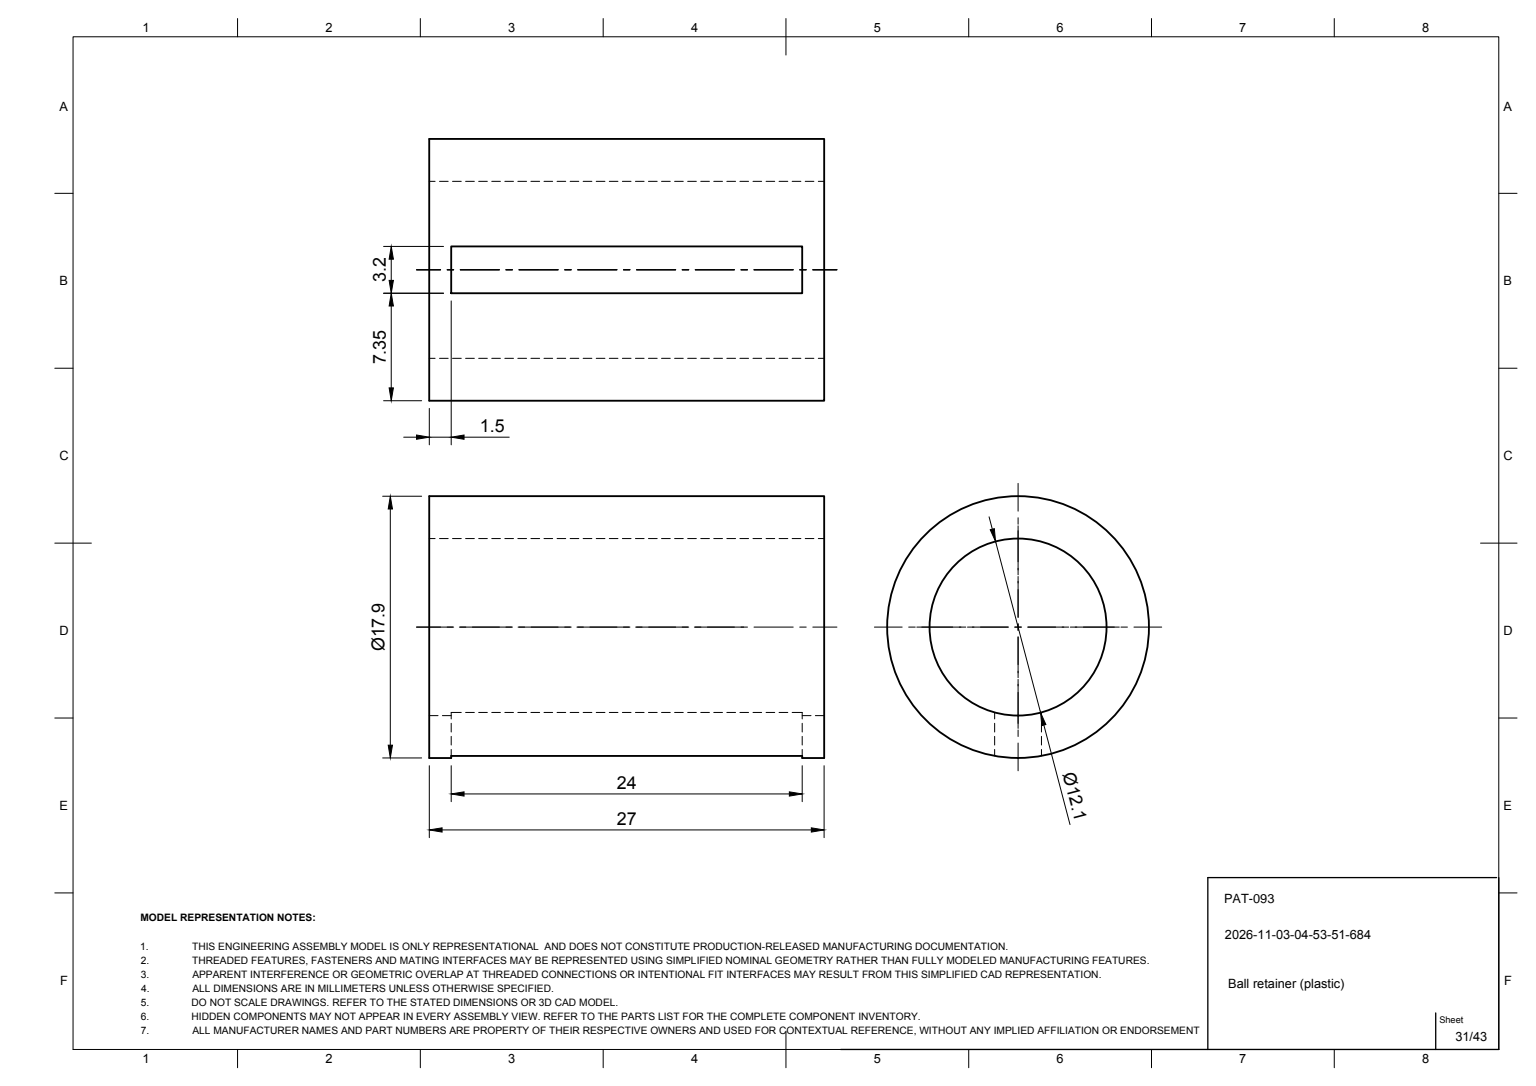
ISO-10303-21;
HEADER;
/* Generated by software containing ST-Developer
 * from STEP Tools, Inc. (www.steptools.com) 
 */

FILE_DESCRIPTION(
/* description */ ('Self-centering screw clamp'),
/* implementation_level */ '2;1');

FILE_NAME(
/* name */ 'Ball retainer (plastic).step',
/* time_stamp */ '2026-10-28T03:25:31-07:00',
/* author */ (''),
/* organization */ (''),
/* preprocessor_version */ 'ST-DEVELOPER v20.2',
/* originating_system */ 'Autodesk Translation Framework v15.17.0.0',
/* authorisation */ '');

FILE_SCHEMA (('AUTOMOTIVE_DESIGN { 1 0 10303 214 3 1 1 }'));
ENDSEC;

DATA;
#10=MECHANICAL_DESIGN_GEOMETRIC_PRESENTATION_REPRESENTATION('',(#661),#16799);
#572=SHAPE_REPRESENTATION_RELATIONSHIP('SRR','None',#17049,#613);
#613=ADVANCED_BREP_SHAPE_REPRESENTATION('',(#709),#16787);
#661=STYLED_ITEM('',(#17319),#709);
#709=MANIFOLD_SOLID_BREP('Body1',#9112);
#988=FACE_BOUND('',#2456,.T.);
#989=FACE_BOUND('',#2458,.T.);
#990=FACE_BOUND('',#2460,.T.);
#991=FACE_BOUND('',#2462,.T.);
#1211=PLANE('',#10462);
#1212=PLANE('',#10465);
#1213=PLANE('',#10466);
#1214=PLANE('',#10469);
#1215=PLANE('',#10470);
#1216=PLANE('',#10475);
#1677=FACE_OUTER_BOUND('',#2451,.T.);
#1678=FACE_OUTER_BOUND('',#2452,.T.);
#1679=FACE_OUTER_BOUND('',#2453,.T.);
#1680=FACE_OUTER_BOUND('',#2454,.T.);
#1681=FACE_OUTER_BOUND('',#2455,.T.);
#1682=FACE_OUTER_BOUND('',#2457,.T.);
#1683=FACE_OUTER_BOUND('',#2459,.T.);
#1684=FACE_OUTER_BOUND('',#2461,.T.);
#2451=EDGE_LOOP('',(#7971,#7972,#7973,#7974));
#2452=EDGE_LOOP('',(#7975,#7976,#7977,#7978));
#2453=EDGE_LOOP('',(#7979,#7980,#7981,#7982));
#2454=EDGE_LOOP('',(#7983,#7984,#7985,#7986));
#2455=EDGE_LOOP('',(#7987));
#2456=EDGE_LOOP('',(#7988));
#2457=EDGE_LOOP('',(#7989,#7990,#7991,#7992));
#2458=EDGE_LOOP('',(#7993,#7994,#7995,#7996));
#2459=EDGE_LOOP('',(#7997));
#2460=EDGE_LOOP('',(#7998));
#2461=EDGE_LOOP('',(#7999,#8000,#8001,#8002));
#2462=EDGE_LOOP('',(#8003,#8004,#8005,#8006));
#3042=LINE('',#16052,#3615);
#3043=LINE('',#16055,#3616);
#3044=LINE('',#16058,#3617);
#3045=LINE('',#16060,#3618);
#3046=LINE('',#16061,#3619);
#3047=LINE('',#16067,#3620);
#3048=LINE('',#16069,#3621);
#3049=LINE('',#16070,#3622);
#3050=LINE('',#16079,#3623);
#3051=LINE('',#16084,#3624);
#3615=VECTOR('',#12991,1.);
#3616=VECTOR('',#12994,1.);
#3617=VECTOR('',#12997,1.);
#3618=VECTOR('',#12998,1.);
#3619=VECTOR('',#12999,1.);
#3620=VECTOR('',#13006,1.);
#3621=VECTOR('',#13009,1.);
#3622=VECTOR('',#13010,1.);
#3623=VECTOR('',#13021,0.895);
#3624=VECTOR('',#13028,0.605);
#4162=CIRCLE('',#10463,0.895);
#4163=CIRCLE('',#10464,0.605);
#4164=CIRCLE('',#10467,0.895);
#4165=CIRCLE('',#10468,0.605);
#4166=CIRCLE('',#10471,0.895);
#4167=CIRCLE('',#10472,0.605);
#4168=CIRCLE('',#10474,0.895);
#4169=CIRCLE('',#10476,0.605);
#4851=VERTEX_POINT('',#16048);
#4852=VERTEX_POINT('',#16049);
#4853=VERTEX_POINT('',#16051);
#4854=VERTEX_POINT('',#16053);
#4855=VERTEX_POINT('',#16057);
#4856=VERTEX_POINT('',#16059);
#4857=VERTEX_POINT('',#16063);
#4858=VERTEX_POINT('',#16065);
#4859=VERTEX_POINT('',#16072);
#4860=VERTEX_POINT('',#16074);
#4861=VERTEX_POINT('',#16077);
#4862=VERTEX_POINT('',#16081);
#5910=EDGE_CURVE('',#4851,#4852,#4162,.T.);
#5911=EDGE_CURVE('',#4853,#4851,#3042,.T.);
#5912=EDGE_CURVE('',#4854,#4853,#4163,.T.);
#5913=EDGE_CURVE('',#4852,#4854,#3043,.T.);
#5914=EDGE_CURVE('',#4852,#4855,#3044,.T.);
#5915=EDGE_CURVE('',#4856,#4854,#3045,.T.);
#5916=EDGE_CURVE('',#4856,#4855,#3046,.T.);
#5917=EDGE_CURVE('',#4855,#4857,#4164,.T.);
#5918=EDGE_CURVE('',#4858,#4856,#4165,.T.);
#5919=EDGE_CURVE('',#4857,#4858,#3047,.T.);
#5920=EDGE_CURVE('',#4857,#4851,#3048,.T.);
#5921=EDGE_CURVE('',#4853,#4858,#3049,.T.);
#5922=EDGE_CURVE('',#4859,#4859,#4166,.T.);
#5923=EDGE_CURVE('',#4860,#4860,#4167,.T.);
#5924=EDGE_CURVE('',#4861,#4861,#4168,.T.);
#5925=EDGE_CURVE('',#4861,#4859,#3050,.T.);
#5926=EDGE_CURVE('',#4862,#4862,#4169,.T.);
#5927=EDGE_CURVE('',#4862,#4860,#3051,.T.);
#7971=ORIENTED_EDGE('',*,*,#5910,.F.);
#7972=ORIENTED_EDGE('',*,*,#5911,.F.);
#7973=ORIENTED_EDGE('',*,*,#5912,.F.);
#7974=ORIENTED_EDGE('',*,*,#5913,.F.);
#7975=ORIENTED_EDGE('',*,*,#5914,.F.);
#7976=ORIENTED_EDGE('',*,*,#5913,.T.);
#7977=ORIENTED_EDGE('',*,*,#5915,.F.);
#7978=ORIENTED_EDGE('',*,*,#5916,.T.);
#7979=ORIENTED_EDGE('',*,*,#5917,.F.);
#7980=ORIENTED_EDGE('',*,*,#5916,.F.);
#7981=ORIENTED_EDGE('',*,*,#5918,.F.);
#7982=ORIENTED_EDGE('',*,*,#5919,.F.);
#7983=ORIENTED_EDGE('',*,*,#5920,.F.);
#7984=ORIENTED_EDGE('',*,*,#5919,.T.);
#7985=ORIENTED_EDGE('',*,*,#5921,.F.);
#7986=ORIENTED_EDGE('',*,*,#5911,.T.);
#7987=ORIENTED_EDGE('',*,*,#5922,.F.);
#7988=ORIENTED_EDGE('',*,*,#5923,.T.);
#7989=ORIENTED_EDGE('',*,*,#5924,.F.);
#7990=ORIENTED_EDGE('',*,*,#5925,.T.);
#7991=ORIENTED_EDGE('',*,*,#5922,.T.);
#7992=ORIENTED_EDGE('',*,*,#5925,.F.);
#7993=ORIENTED_EDGE('',*,*,#5917,.T.);
#7994=ORIENTED_EDGE('',*,*,#5920,.T.);
#7995=ORIENTED_EDGE('',*,*,#5910,.T.);
#7996=ORIENTED_EDGE('',*,*,#5914,.T.);
#7997=ORIENTED_EDGE('',*,*,#5924,.T.);
#7998=ORIENTED_EDGE('',*,*,#5926,.F.);
#7999=ORIENTED_EDGE('',*,*,#5926,.T.);
#8000=ORIENTED_EDGE('',*,*,#5927,.T.);
#8001=ORIENTED_EDGE('',*,*,#5923,.F.);
#8002=ORIENTED_EDGE('',*,*,#5927,.F.);
#8003=ORIENTED_EDGE('',*,*,#5918,.T.);
#8004=ORIENTED_EDGE('',*,*,#5915,.T.);
#8005=ORIENTED_EDGE('',*,*,#5912,.T.);
#8006=ORIENTED_EDGE('',*,*,#5921,.T.);
#8542=CYLINDRICAL_SURFACE('',#10473,0.895);
#8543=CYLINDRICAL_SURFACE('',#10477,0.605);
#8975=ADVANCED_FACE('',(#1677),#1211,.F.);
#8976=ADVANCED_FACE('',(#1678),#1212,.F.);
#8977=ADVANCED_FACE('',(#1679),#1213,.F.);
#8978=ADVANCED_FACE('',(#1680),#1214,.F.);
#8979=ADVANCED_FACE('',(#1681,#988),#1215,.T.);
#8980=ADVANCED_FACE('',(#1682,#989),#8542,.T.);
#8981=ADVANCED_FACE('',(#1683,#990),#1216,.T.);
#8982=ADVANCED_FACE('',(#1684,#991),#8543,.F.);
#9112=CLOSED_SHELL('',(#8975,#8976,#8977,#8978,#8979,#8980,#8981,#8982));
#10461=AXIS2_PLACEMENT_3D('',#16046,#12985,#12986);
#10462=AXIS2_PLACEMENT_3D('',#16047,#12987,#12988);
#10463=AXIS2_PLACEMENT_3D('',#16050,#12989,#12990);
#10464=AXIS2_PLACEMENT_3D('',#16054,#12992,#12993);
#10465=AXIS2_PLACEMENT_3D('',#16056,#12995,#12996);
#10466=AXIS2_PLACEMENT_3D('',#16062,#13000,#13001);
#10467=AXIS2_PLACEMENT_3D('',#16064,#13002,#13003);
#10468=AXIS2_PLACEMENT_3D('',#16066,#13004,#13005);
#10469=AXIS2_PLACEMENT_3D('',#16068,#13007,#13008);
#10470=AXIS2_PLACEMENT_3D('',#16071,#13011,#13012);
#10471=AXIS2_PLACEMENT_3D('',#16073,#13013,#13014);
#10472=AXIS2_PLACEMENT_3D('',#16075,#13015,#13016);
#10473=AXIS2_PLACEMENT_3D('',#16076,#13017,#13018);
#10474=AXIS2_PLACEMENT_3D('',#16078,#13019,#13020);
#10475=AXIS2_PLACEMENT_3D('',#16080,#13022,#13023);
#10476=AXIS2_PLACEMENT_3D('',#16082,#13024,#13025);
#10477=AXIS2_PLACEMENT_3D('',#16083,#13026,#13027);
#12985=DIRECTION('axis',(0.,0.,1.));
#12986=DIRECTION('refdir',(1.,0.,0.));
#12987=DIRECTION('center_axis',(0.,1.,0.));
#12988=DIRECTION('ref_axis',(0.,0.,1.));
#12989=DIRECTION('center_axis',(0.,1.,0.));
#12990=DIRECTION('ref_axis',(1.,0.,0.));
#12991=DIRECTION('',(1.,0.,0.));
#12992=DIRECTION('center_axis',(0.,-1.,0.));
#12993=DIRECTION('ref_axis',(1.,0.,0.));
#12994=DIRECTION('',(-1.,0.,0.));
#12995=DIRECTION('center_axis',(0.,0.,-1.));
#12996=DIRECTION('ref_axis',(-1.,0.,0.));
#12997=DIRECTION('',(0.,-1.,0.));
#12998=DIRECTION('',(0.,1.,0.));
#12999=DIRECTION('',(1.,0.,0.));
#13000=DIRECTION('center_axis',(0.,-1.,0.));
#13001=DIRECTION('ref_axis',(0.,0.,-1.));
#13002=DIRECTION('center_axis',(0.,-1.,0.));
#13003=DIRECTION('ref_axis',(1.,0.,0.));
#13004=DIRECTION('center_axis',(0.,1.,0.));
#13005=DIRECTION('ref_axis',(1.,0.,0.));
#13006=DIRECTION('',(-1.,0.,0.));
#13007=DIRECTION('center_axis',(0.,0.,1.));
#13008=DIRECTION('ref_axis',(1.,0.,0.));
#13009=DIRECTION('',(0.,1.,0.));
#13010=DIRECTION('',(0.,-1.,0.));
#13011=DIRECTION('center_axis',(0.,1.,0.));
#13012=DIRECTION('ref_axis',(0.,0.,1.));
#13013=DIRECTION('center_axis',(0.,-1.,0.));
#13014=DIRECTION('ref_axis',(1.,0.,0.));
#13015=DIRECTION('center_axis',(0.,-1.,0.));
#13016=DIRECTION('ref_axis',(1.,0.,0.));
#13017=DIRECTION('center_axis',(0.,-1.,0.));
#13018=DIRECTION('ref_axis',(1.,0.,0.));
#13019=DIRECTION('center_axis',(0.,-1.,0.));
#13020=DIRECTION('ref_axis',(1.,0.,0.));
#13021=DIRECTION('',(0.,1.,0.));
#13022=DIRECTION('center_axis',(0.,-1.,0.));
#13023=DIRECTION('ref_axis',(0.,0.,-1.));
#13024=DIRECTION('center_axis',(0.,-1.,0.));
#13025=DIRECTION('ref_axis',(1.,0.,0.));
#13026=DIRECTION('center_axis',(0.,-1.,0.));
#13027=DIRECTION('ref_axis',(1.,0.,0.));
#13028=DIRECTION('',(0.,1.,0.));
#16046=CARTESIAN_POINT('',(0.,0.,0.));
#16047=CARTESIAN_POINT('Origin',(0.75,1.2,0.));
#16048=CARTESIAN_POINT('',(0.880582193778639,1.2,0.16));
#16049=CARTESIAN_POINT('',(0.880582193778639,1.2,-0.16));
#16050=CARTESIAN_POINT('Origin',(0.,1.2,0.));
#16051=CARTESIAN_POINT('',(0.583459510163302,1.2,0.16));
#16052=CARTESIAN_POINT('',(0.57,1.2,0.16));
#16053=CARTESIAN_POINT('',(0.583459510163302,1.2,-0.16));
#16054=CARTESIAN_POINT('Origin',(0.,1.2,0.));
#16055=CARTESIAN_POINT('',(0.93,1.2,-0.16));
#16056=CARTESIAN_POINT('Origin',(0.93,0.,-0.16));
#16057=CARTESIAN_POINT('',(0.880582193778639,-1.2,-0.16));
#16058=CARTESIAN_POINT('',(0.880582193778639,0.,-0.16));
#16059=CARTESIAN_POINT('',(0.583459510163302,-1.2,-0.16));
#16060=CARTESIAN_POINT('',(0.583459510163302,0.,-0.16));
#16061=CARTESIAN_POINT('',(0.93,-1.2,-0.16));
#16062=CARTESIAN_POINT('Origin',(0.75,-1.2,0.));
#16063=CARTESIAN_POINT('',(0.880582193778639,-1.2,0.16));
#16064=CARTESIAN_POINT('Origin',(0.,-1.2,0.));
#16065=CARTESIAN_POINT('',(0.583459510163302,-1.2,0.16));
#16066=CARTESIAN_POINT('Origin',(0.,-1.2,0.));
#16067=CARTESIAN_POINT('',(0.57,-1.2,0.16));
#16068=CARTESIAN_POINT('Origin',(0.57,0.,0.16));
#16069=CARTESIAN_POINT('',(0.880582193778639,0.,0.16));
#16070=CARTESIAN_POINT('',(0.583459510163302,0.,0.16));
#16071=CARTESIAN_POINT('Origin',(0.895,1.35,0.));
#16072=CARTESIAN_POINT('',(-0.895,1.35,-1.09605888523688E-16));
#16073=CARTESIAN_POINT('Origin',(0.,1.35,0.));
#16074=CARTESIAN_POINT('',(-0.605,1.35,-7.40911313484149E-17));
#16075=CARTESIAN_POINT('Origin',(0.,1.35,0.));
#16076=CARTESIAN_POINT('Origin',(0.,0.,0.));
#16077=CARTESIAN_POINT('',(-0.895,-1.35,-1.09605888523688E-16));
#16078=CARTESIAN_POINT('Origin',(0.,-1.35,0.));
#16079=CARTESIAN_POINT('',(-0.895,0.,-1.09605888523688E-16));
#16080=CARTESIAN_POINT('Origin',(0.605,-1.35,0.));
#16081=CARTESIAN_POINT('',(-0.605,-1.35,-7.40911313484149E-17));
#16082=CARTESIAN_POINT('Origin',(0.,-1.35,0.));
#16083=CARTESIAN_POINT('Origin',(0.,0.,0.));
#16084=CARTESIAN_POINT('',(-0.605,0.,-7.40911313484149E-17));
#16738=UNCERTAINTY_MEASURE_WITH_UNIT(LENGTH_MEASURE(0.001),#16800,
'DISTANCE_ACCURACY_VALUE',
'Maximum model space distance between geometric entities at asserted c
onnectivities');
#16750=UNCERTAINTY_MEASURE_WITH_UNIT(LENGTH_MEASURE(0.001),#16800,
'DISTANCE_ACCURACY_VALUE',
'Maximum model space distance between geometric entities at asserted c
onnectivities');
#16787=(
GEOMETRIC_REPRESENTATION_CONTEXT(3)
GLOBAL_UNCERTAINTY_ASSIGNED_CONTEXT((#16738))
GLOBAL_UNIT_ASSIGNED_CONTEXT((#16800,#16802,#16803))
REPRESENTATION_CONTEXT('','3D')
);
#16799=(
GEOMETRIC_REPRESENTATION_CONTEXT(3)
GLOBAL_UNCERTAINTY_ASSIGNED_CONTEXT((#16750))
GLOBAL_UNIT_ASSIGNED_CONTEXT((#16800,#16802,#16803))
REPRESENTATION_CONTEXT('','3D')
);
#16800=(
LENGTH_UNIT()
NAMED_UNIT(*)
SI_UNIT(.CENTI.,.METRE.)
);
#16802=(
NAMED_UNIT(*)
PLANE_ANGLE_UNIT()
SI_UNIT($,.RADIAN.)
);
#16803=(
NAMED_UNIT(*)
SI_UNIT($,.STERADIAN.)
SOLID_ANGLE_UNIT()
);
#16840=SHAPE_DEFINITION_REPRESENTATION(#16893,#17049);
#16893=PRODUCT_DEFINITION_SHAPE('',$,#17098);
#17049=SHAPE_REPRESENTATION('',(#10461),#16787);
#17061=PRODUCT_DEFINITION_CONTEXT('part definition',#17207,'design');
#17098=PRODUCT_DEFINITION('Ball retainer (plastic)',
'Ball retainer (plastic)',#17146,#17061);
#17146=PRODUCT_DEFINITION_FORMATION('',$,#17245);
#17207=APPLICATION_CONTEXT(
'Core Data for Automotive Mechanical Design Process');
#17208=PRODUCT_CONTEXT('part definition',#17207,'mechanical');
#17245=PRODUCT('Ball retainer (plastic)','Ball retainer (plastic)',
'Ball retainer (plastic)',(#17208));
#17313=COLOUR_RGB('Sky Blue',0.24,0.69,0.87);
#17314=FILL_AREA_STYLE_COLOUR('',#17313);
#17315=FILL_AREA_STYLE('',(#17314));
#17316=SURFACE_STYLE_FILL_AREA(#17315);
#17317=SURFACE_SIDE_STYLE('',(#17316));
#17318=SURFACE_STYLE_USAGE(.BOTH.,#17317);
#17319=PRESENTATION_STYLE_ASSIGNMENT((#17318));
ENDSEC;
END-ISO-10303-21;
